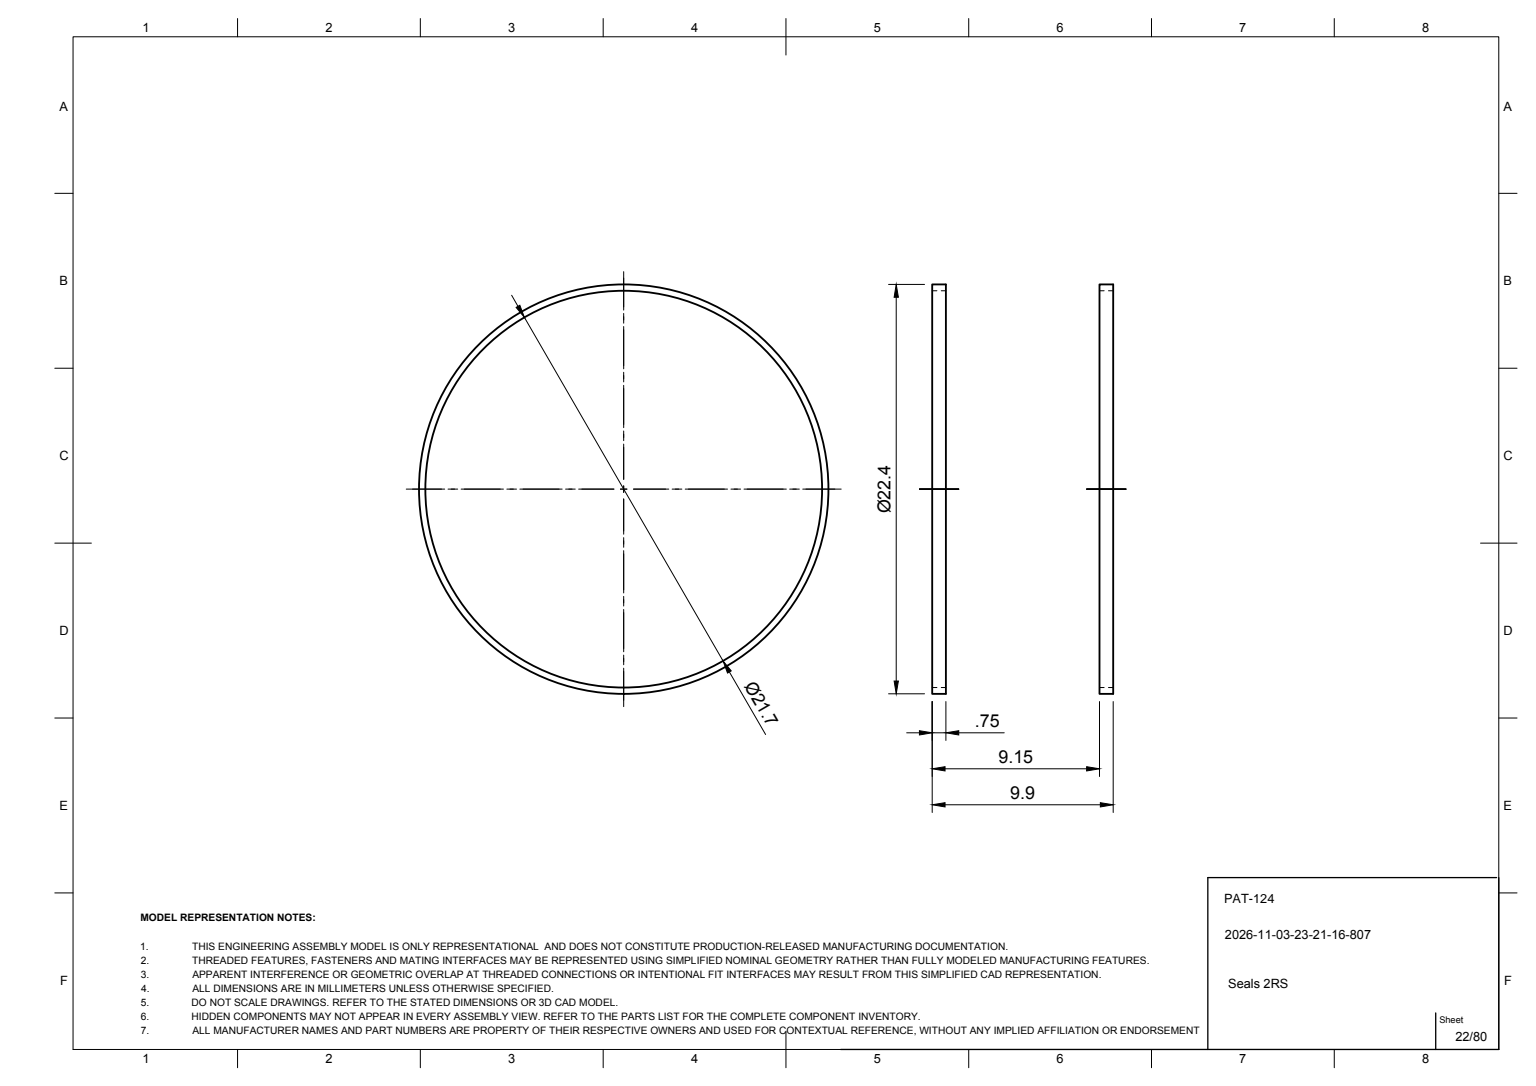
ISO-10303-21;
HEADER;
/* Generated by software containing ST-Developer
 * from STEP Tools, Inc. (www.steptools.com) 
 */

FILE_DESCRIPTION(
/* description */ ('XY cross-slide table'),
/* implementation_level */ '2;1');

FILE_NAME(
/* name */ 'Seals 2RS.step',
/* time_stamp */ '2026-10-28T03:22:46-07:00',
/* author */ (''),
/* organization */ (''),
/* preprocessor_version */ 'ST-DEVELOPER v20.2',
/* originating_system */ 'Autodesk Translation Framework v15.17.0.0',
/* authorisation */ '');

FILE_SCHEMA (('AUTOMOTIVE_DESIGN { 1 0 10303 214 3 1 1 }'));
ENDSEC;

DATA;
#10=MECHANICAL_DESIGN_GEOMETRIC_PRESENTATION_REPRESENTATION('',(#1691,#1692),#62984);
#1519=SHAPE_REPRESENTATION_RELATIONSHIP('SRR','None',#63368,#1602);
#1602=ADVANCED_BREP_SHAPE_REPRESENTATION('',(#1804,#1805),#62905);
#1691=STYLED_ITEM('',(#63912),#1804);
#1692=STYLED_ITEM('',(#63912),#1805);
#1804=MANIFOLD_SOLID_BREP('Body1',#22985);
#1805=MANIFOLD_SOLID_BREP('Body2',#22986);
#1988=FACE_BOUND('',#4472,.T.);
#1989=FACE_BOUND('',#4475,.T.);
#1990=FACE_BOUND('',#4478,.T.);
#1991=FACE_BOUND('',#4481,.T.);
#2393=PLANE('',#24392);
#2394=PLANE('',#24397);
#2395=PLANE('',#24400);
#2396=PLANE('',#24405);
#3056=FACE_OUTER_BOUND('',#4471,.T.);
#3057=FACE_OUTER_BOUND('',#4473,.T.);
#3058=FACE_OUTER_BOUND('',#4474,.T.);
#3059=FACE_OUTER_BOUND('',#4476,.T.);
#3060=FACE_OUTER_BOUND('',#4477,.T.);
#3061=FACE_OUTER_BOUND('',#4479,.T.);
#3062=FACE_OUTER_BOUND('',#4480,.T.);
#3063=FACE_OUTER_BOUND('',#4482,.T.);
#4471=EDGE_LOOP('',(#15728));
#4472=EDGE_LOOP('',(#15729));
#4473=EDGE_LOOP('',(#15730,#15731,#15732,#15733));
#4474=EDGE_LOOP('',(#15734));
#4475=EDGE_LOOP('',(#15735));
#4476=EDGE_LOOP('',(#15736,#15737,#15738,#15739));
#4477=EDGE_LOOP('',(#15740));
#4478=EDGE_LOOP('',(#15741));
#4479=EDGE_LOOP('',(#15742,#15743,#15744,#15745));
#4480=EDGE_LOOP('',(#15746));
#4481=EDGE_LOOP('',(#15747));
#4482=EDGE_LOOP('',(#15748,#15749,#15750,#15751));
#6119=LINE('',#34071,#7606);
#6120=LINE('',#34076,#7607);
#6121=LINE('',#34085,#7608);
#6122=LINE('',#34090,#7609);
#7606=VECTOR('',#27468,1.119765);
#7607=VECTOR('',#27475,1.085235);
#7608=VECTOR('',#27486,1.119765);
#7609=VECTOR('',#27493,1.085235);
#9065=CIRCLE('',#24393,1.119765);
#9066=CIRCLE('',#24394,1.085235);
#9067=CIRCLE('',#24396,1.119765);
#9068=CIRCLE('',#24398,1.085235);
#9069=CIRCLE('',#24401,1.119765);
#9070=CIRCLE('',#24402,1.085235);
#9071=CIRCLE('',#24404,1.119765);
#9072=CIRCLE('',#24406,1.085235);
#10053=VERTEX_POINT('',#34064);
#10054=VERTEX_POINT('',#34066);
#10055=VERTEX_POINT('',#34069);
#10056=VERTEX_POINT('',#34073);
#10057=VERTEX_POINT('',#34078);
#10058=VERTEX_POINT('',#34080);
#10059=VERTEX_POINT('',#34083);
#10060=VERTEX_POINT('',#34087);
#12248=EDGE_CURVE('',#10053,#10053,#9065,.T.);
#12249=EDGE_CURVE('',#10054,#10054,#9066,.T.);
#12250=EDGE_CURVE('',#10055,#10055,#9067,.T.);
#12251=EDGE_CURVE('',#10055,#10053,#6119,.T.);
#12252=EDGE_CURVE('',#10056,#10056,#9068,.T.);
#12253=EDGE_CURVE('',#10056,#10054,#6120,.T.);
#12254=EDGE_CURVE('',#10057,#10057,#9069,.T.);
#12255=EDGE_CURVE('',#10058,#10058,#9070,.T.);
#12256=EDGE_CURVE('',#10059,#10059,#9071,.T.);
#12257=EDGE_CURVE('',#10059,#10057,#6121,.T.);
#12258=EDGE_CURVE('',#10060,#10060,#9072,.T.);
#12259=EDGE_CURVE('',#10060,#10058,#6122,.T.);
#15728=ORIENTED_EDGE('',*,*,#12248,.F.);
#15729=ORIENTED_EDGE('',*,*,#12249,.T.);
#15730=ORIENTED_EDGE('',*,*,#12250,.F.);
#15731=ORIENTED_EDGE('',*,*,#12251,.T.);
#15732=ORIENTED_EDGE('',*,*,#12248,.T.);
#15733=ORIENTED_EDGE('',*,*,#12251,.F.);
#15734=ORIENTED_EDGE('',*,*,#12250,.T.);
#15735=ORIENTED_EDGE('',*,*,#12252,.F.);
#15736=ORIENTED_EDGE('',*,*,#12252,.T.);
#15737=ORIENTED_EDGE('',*,*,#12253,.T.);
#15738=ORIENTED_EDGE('',*,*,#12249,.F.);
#15739=ORIENTED_EDGE('',*,*,#12253,.F.);
#15740=ORIENTED_EDGE('',*,*,#12254,.F.);
#15741=ORIENTED_EDGE('',*,*,#12255,.T.);
#15742=ORIENTED_EDGE('',*,*,#12256,.F.);
#15743=ORIENTED_EDGE('',*,*,#12257,.T.);
#15744=ORIENTED_EDGE('',*,*,#12254,.T.);
#15745=ORIENTED_EDGE('',*,*,#12257,.F.);
#15746=ORIENTED_EDGE('',*,*,#12256,.T.);
#15747=ORIENTED_EDGE('',*,*,#12258,.F.);
#15748=ORIENTED_EDGE('',*,*,#12258,.T.);
#15749=ORIENTED_EDGE('',*,*,#12259,.T.);
#15750=ORIENTED_EDGE('',*,*,#12255,.F.);
#15751=ORIENTED_EDGE('',*,*,#12259,.F.);
#21110=CYLINDRICAL_SURFACE('',#24395,1.119765);
#21111=CYLINDRICAL_SURFACE('',#24399,1.085235);
#21112=CYLINDRICAL_SURFACE('',#24403,1.119765);
#21113=CYLINDRICAL_SURFACE('',#24407,1.085235);
#21837=ADVANCED_FACE('',(#3056,#1988),#2393,.T.);
#21838=ADVANCED_FACE('',(#3057),#21110,.T.);
#21839=ADVANCED_FACE('',(#3058,#1989),#2394,.T.);
#21840=ADVANCED_FACE('',(#3059),#21111,.F.);
#21841=ADVANCED_FACE('',(#3060,#1990),#2395,.T.);
#21842=ADVANCED_FACE('',(#3061),#21112,.T.);
#21843=ADVANCED_FACE('',(#3062,#1991),#2396,.T.);
#21844=ADVANCED_FACE('',(#3063),#21113,.F.);
#22985=CLOSED_SHELL('',(#21837,#21838,#21839,#21840));
#22986=CLOSED_SHELL('',(#21841,#21842,#21843,#21844));
#24391=AXIS2_PLACEMENT_3D('',#34062,#27456,#27457);
#24392=AXIS2_PLACEMENT_3D('',#34063,#27458,#27459);
#24393=AXIS2_PLACEMENT_3D('',#34065,#27460,#27461);
#24394=AXIS2_PLACEMENT_3D('',#34067,#27462,#27463);
#24395=AXIS2_PLACEMENT_3D('',#34068,#27464,#27465);
#24396=AXIS2_PLACEMENT_3D('',#34070,#27466,#27467);
#24397=AXIS2_PLACEMENT_3D('',#34072,#27469,#27470);
#24398=AXIS2_PLACEMENT_3D('',#34074,#27471,#27472);
#24399=AXIS2_PLACEMENT_3D('',#34075,#27473,#27474);
#24400=AXIS2_PLACEMENT_3D('',#34077,#27476,#27477);
#24401=AXIS2_PLACEMENT_3D('',#34079,#27478,#27479);
#24402=AXIS2_PLACEMENT_3D('',#34081,#27480,#27481);
#24403=AXIS2_PLACEMENT_3D('',#34082,#27482,#27483);
#24404=AXIS2_PLACEMENT_3D('',#34084,#27484,#27485);
#24405=AXIS2_PLACEMENT_3D('',#34086,#27487,#27488);
#24406=AXIS2_PLACEMENT_3D('',#34088,#27489,#27490);
#24407=AXIS2_PLACEMENT_3D('',#34089,#27491,#27492);
#27456=DIRECTION('axis',(0.,0.,1.));
#27457=DIRECTION('refdir',(1.,0.,0.));
#27458=DIRECTION('center_axis',(0.,1.,0.));
#27459=DIRECTION('ref_axis',(0.,0.,1.));
#27460=DIRECTION('center_axis',(0.,-1.,0.));
#27461=DIRECTION('ref_axis',(1.,0.,0.));
#27462=DIRECTION('center_axis',(0.,-1.,0.));
#27463=DIRECTION('ref_axis',(1.,0.,0.));
#27464=DIRECTION('center_axis',(0.,-1.,0.));
#27465=DIRECTION('ref_axis',(1.,0.,0.));
#27466=DIRECTION('center_axis',(0.,-1.,0.));
#27467=DIRECTION('ref_axis',(1.,0.,0.));
#27468=DIRECTION('',(0.,1.,0.));
#27469=DIRECTION('center_axis',(0.,-1.,0.));
#27470=DIRECTION('ref_axis',(0.,0.,-1.));
#27471=DIRECTION('center_axis',(0.,-1.,0.));
#27472=DIRECTION('ref_axis',(1.,0.,0.));
#27473=DIRECTION('center_axis',(0.,-1.,0.));
#27474=DIRECTION('ref_axis',(1.,0.,0.));
#27475=DIRECTION('',(0.,1.,0.));
#27476=DIRECTION('center_axis',(0.,1.,0.));
#27477=DIRECTION('ref_axis',(0.,0.,1.));
#27478=DIRECTION('center_axis',(0.,-1.,0.));
#27479=DIRECTION('ref_axis',(1.,0.,0.));
#27480=DIRECTION('center_axis',(0.,-1.,0.));
#27481=DIRECTION('ref_axis',(1.,0.,0.));
#27482=DIRECTION('center_axis',(0.,-1.,0.));
#27483=DIRECTION('ref_axis',(1.,0.,0.));
#27484=DIRECTION('center_axis',(0.,-1.,0.));
#27485=DIRECTION('ref_axis',(1.,0.,0.));
#27486=DIRECTION('',(0.,1.,0.));
#27487=DIRECTION('center_axis',(0.,-1.,0.));
#27488=DIRECTION('ref_axis',(0.,0.,-1.));
#27489=DIRECTION('center_axis',(0.,-1.,0.));
#27490=DIRECTION('ref_axis',(1.,0.,0.));
#27491=DIRECTION('center_axis',(0.,-1.,0.));
#27492=DIRECTION('ref_axis',(1.,0.,0.));
#27493=DIRECTION('',(0.,1.,0.));
#34062=CARTESIAN_POINT('',(0.,0.,0.));
#34063=CARTESIAN_POINT('Origin',(1.119765,0.495,0.));
#34064=CARTESIAN_POINT('',(-1.119765,0.495,-1.37131662304724E-16));
#34065=CARTESIAN_POINT('Origin',(0.,0.495,0.));
#34066=CARTESIAN_POINT('',(-1.085235,0.495,-1.32902956907268E-16));
#34067=CARTESIAN_POINT('Origin',(0.,0.495,0.));
#34068=CARTESIAN_POINT('Origin',(0.,0.4575,0.));
#34069=CARTESIAN_POINT('',(-1.119765,0.42,-1.37131662304724E-16));
#34070=CARTESIAN_POINT('Origin',(0.,0.42,0.));
#34071=CARTESIAN_POINT('',(-1.119765,0.4575,-1.37131662304724E-16));
#34072=CARTESIAN_POINT('Origin',(1.085235,0.42,0.));
#34073=CARTESIAN_POINT('',(-1.085235,0.42,-1.32902956907268E-16));
#34074=CARTESIAN_POINT('Origin',(0.,0.42,0.));
#34075=CARTESIAN_POINT('Origin',(0.,0.4575,0.));
#34076=CARTESIAN_POINT('',(-1.085235,0.4575,-1.32902956907268E-16));
#34077=CARTESIAN_POINT('Origin',(1.119765,-0.42,0.));
#34078=CARTESIAN_POINT('',(-1.119765,-0.42,-1.37131662304724E-16));
#34079=CARTESIAN_POINT('Origin',(0.,-0.42,0.));
#34080=CARTESIAN_POINT('',(-1.085235,-0.42,-1.32902956907268E-16));
#34081=CARTESIAN_POINT('Origin',(0.,-0.42,0.));
#34082=CARTESIAN_POINT('Origin',(0.,-0.4575,0.));
#34083=CARTESIAN_POINT('',(-1.119765,-0.495,-1.37131662304724E-16));
#34084=CARTESIAN_POINT('Origin',(0.,-0.495,0.));
#34085=CARTESIAN_POINT('',(-1.119765,-0.4575,-1.37131662304724E-16));
#34086=CARTESIAN_POINT('Origin',(1.085235,-0.495,0.));
#34087=CARTESIAN_POINT('',(-1.085235,-0.495,-1.32902956907268E-16));
#34088=CARTESIAN_POINT('Origin',(0.,-0.495,0.));
#34089=CARTESIAN_POINT('Origin',(0.,-0.4575,0.));
#34090=CARTESIAN_POINT('',(-1.085235,-0.4575,-1.32902956907268E-16));
#62806=UNCERTAINTY_MEASURE_WITH_UNIT(LENGTH_MEASURE(0.001),#62985,
'DISTANCE_ACCURACY_VALUE',
'Maximum model space distance between geometric entities at asserted c
onnectivities');
#62885=UNCERTAINTY_MEASURE_WITH_UNIT(LENGTH_MEASURE(0.001),#62985,
'DISTANCE_ACCURACY_VALUE',
'Maximum model space distance between geometric entities at asserted c
onnectivities');
#62905=(
GEOMETRIC_REPRESENTATION_CONTEXT(3)
GLOBAL_UNCERTAINTY_ASSIGNED_CONTEXT((#62806))
GLOBAL_UNIT_ASSIGNED_CONTEXT((#62985,#62987,#62988))
REPRESENTATION_CONTEXT('','3D')
);
#62984=(
GEOMETRIC_REPRESENTATION_CONTEXT(3)
GLOBAL_UNCERTAINTY_ASSIGNED_CONTEXT((#62885))
GLOBAL_UNIT_ASSIGNED_CONTEXT((#62985,#62987,#62988))
REPRESENTATION_CONTEXT('','3D')
);
#62985=(
LENGTH_UNIT()
NAMED_UNIT(*)
SI_UNIT(.CENTI.,.METRE.)
);
#62987=(
NAMED_UNIT(*)
PLANE_ANGLE_UNIT()
SI_UNIT($,.RADIAN.)
);
#62988=(
NAMED_UNIT(*)
SI_UNIT($,.STERADIAN.)
SOLID_ANGLE_UNIT()
);
#63008=SHAPE_DEFINITION_REPRESENTATION(#63106,#63368);
#63106=PRODUCT_DEFINITION_SHAPE('',$,#63467);
#63368=SHAPE_REPRESENTATION('',(#24391),#62905);
#63447=PRODUCT_DEFINITION_CONTEXT('part definition',#63743,'design');
#63467=PRODUCT_DEFINITION('Seals 2RS','Seals 2RS',#63565,#63447);
#63565=PRODUCT_DEFINITION_FORMATION('',$,#63764);
#63743=APPLICATION_CONTEXT(
'Core Data for Automotive Mechanical Design Process');
#63744=PRODUCT_CONTEXT('part definition',#63743,'mechanical');
#63764=PRODUCT('Seals 2RS','Seals 2RS','Seals 2RS',(#63744));
#63906=COLOUR_RGB('Grey',0.48,0.52,0.57);
#63907=FILL_AREA_STYLE_COLOUR('',#63906);
#63908=FILL_AREA_STYLE('',(#63907));
#63909=SURFACE_STYLE_FILL_AREA(#63908);
#63910=SURFACE_SIDE_STYLE('',(#63909));
#63911=SURFACE_STYLE_USAGE(.BOTH.,#63910);
#63912=PRESENTATION_STYLE_ASSIGNMENT((#63911));
ENDSEC;
END-ISO-10303-21;
